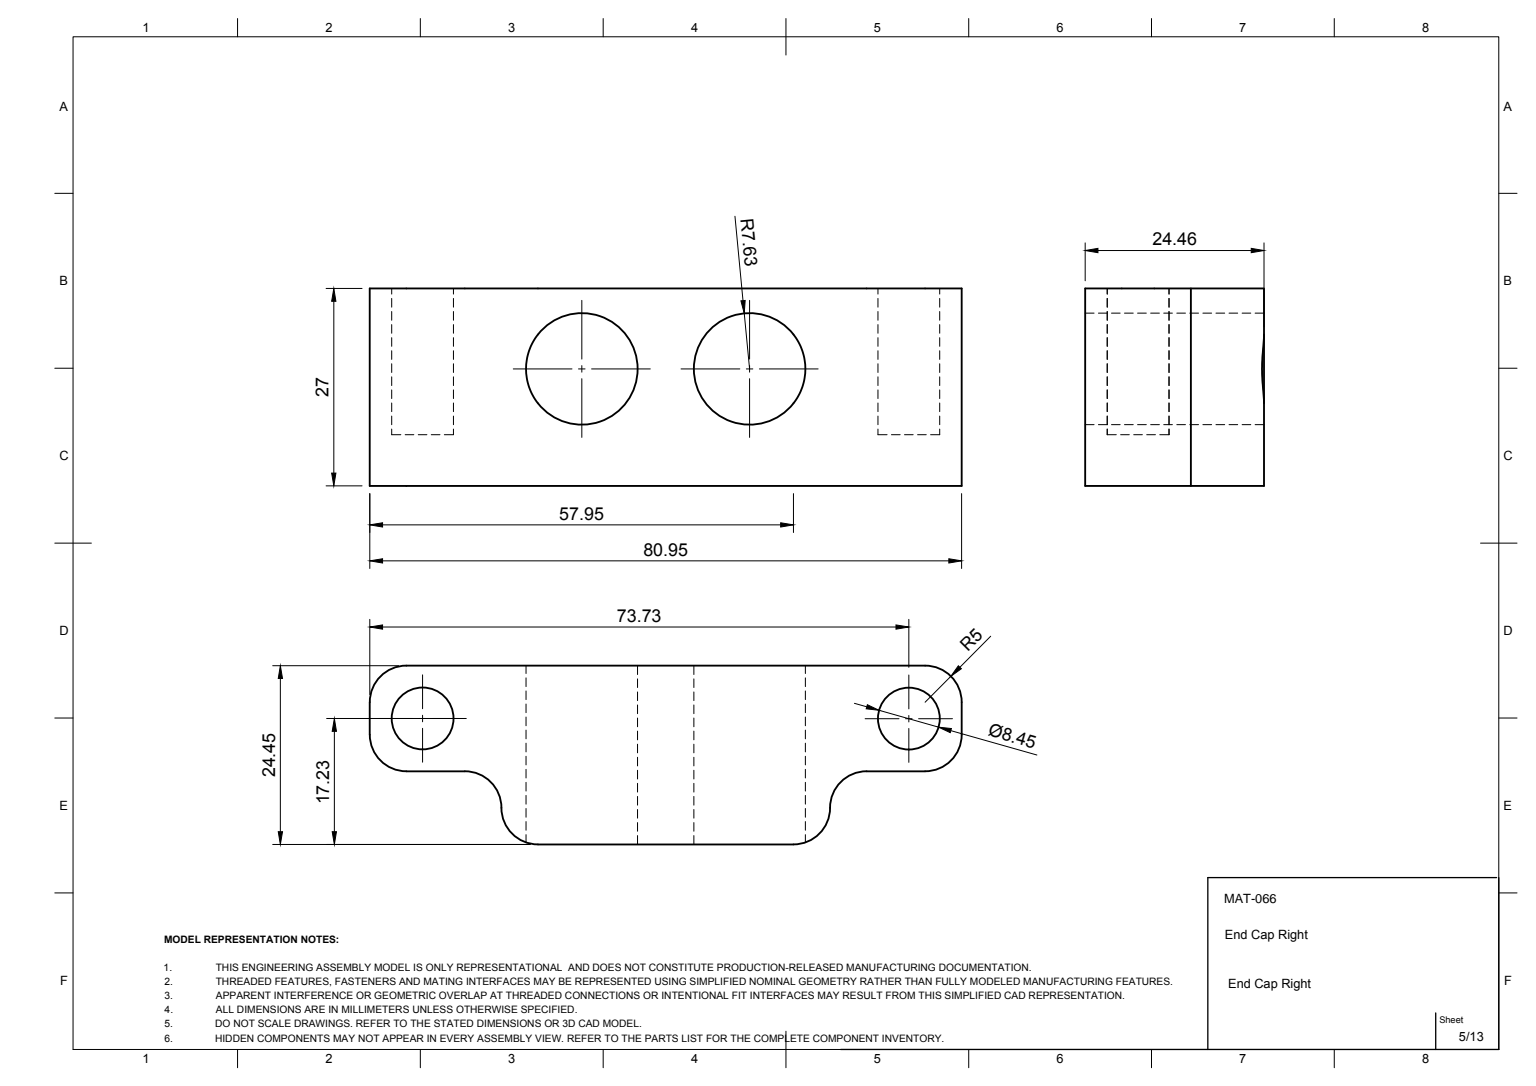
ISO-10303-21;
HEADER;
/* Generated by software containing ST-Developer
 * from STEP Tools, Inc. (www.steptools.com) 
 */

FILE_DESCRIPTION(
/* description */ ('CAx-IF Rec.Pracs.---Representation and Presentation of Product Manufa
cturing Information (PMI)---4.0---2014-10-13'),
/* implementation_level */ '2;1');

FILE_NAME(
/* name */ 'End Cap Right.step',
/* time_stamp */ '2026-10-24T15:58:00-07:00',
/* author */ (''),
/* organization */ (''),
/* preprocessor_version */ 'ST-DEVELOPER v20.2',
/* originating_system */ 'Autodesk Translation Framework v15.17.0.0',
/* authorisation */ '');

FILE_SCHEMA (('AP242_MANAGED_MODEL_BASED_3D_ENGINEERING_MIM_LF { 1 0 10303 442 2 1 4 }'));
ENDSEC;

DATA;
#10=MECHANICAL_DESIGN_GEOMETRIC_PRESENTATION_REPRESENTATION('',(#131),#8944);
#113=SHAPE_REPRESENTATION_RELATIONSHIP('SRR','None',#8995,#122);
#122=ADVANCED_BREP_SHAPE_REPRESENTATION('',(#140),#8936);
#131=STYLED_ITEM('',(#9054),#140);
#140=MANIFOLD_SOLID_BREP('Body1',#5152);
#150=B_SPLINE_CURVE_WITH_KNOTS('',3,(#8654,#8655,#8656,#8657,#8658,#8659),
 .UNSPECIFIED.,.F.,.F.,(4,2,4),(3.46797062946804,3.66737221611079,3.95578831781598),
 .UNSPECIFIED.);
#151=B_SPLINE_CURVE_WITH_KNOTS('',3,(#8660,#8661,#8662,#8663,#8664,#8665),
 .UNSPECIFIED.,.F.,.F.,(4,2,4),(3.95578831781598,4.24420441952117,4.44360600616391),
 .UNSPECIFIED.);
#152=B_SPLINE_CURVE_WITH_KNOTS('',3,(#8668,#8669,#8670,#8671,#8672,#8673,
#8674,#8675,#8676,#8677),.UNSPECIFIED.,.F.,.F.,(4,2,2,2,4),(3.46797062946804,
3.66737221611078,3.95578831781597,4.24420441952117,4.44360600616391),
 .UNSPECIFIED.);
#205=CYLINDRICAL_SURFACE('',#5639,0.004225);
#206=CYLINDRICAL_SURFACE('',#5643,0.004225);
#207=CYLINDRICAL_SURFACE('',#5657,0.005);
#208=CYLINDRICAL_SURFACE('',#5658,0.005);
#209=CYLINDRICAL_SURFACE('',#5659,0.005);
#210=CYLINDRICAL_SURFACE('',#5660,0.005);
#211=CYLINDRICAL_SURFACE('',#5665,0.007625);
#212=CYLINDRICAL_SURFACE('',#5666,0.007625);
#213=CYLINDRICAL_SURFACE('',#5667,0.005);
#214=CYLINDRICAL_SURFACE('',#5668,0.005);
#215=CYLINDRICAL_SURFACE('',#5669,0.005);
#216=CYLINDRICAL_SURFACE('',#5670,0.005);
#284=FACE_BOUND('',#819,.T.);
#285=FACE_BOUND('',#820,.T.);
#286=FACE_BOUND('',#826,.T.);
#287=FACE_BOUND('',#827,.T.);
#500=FACE_OUTER_BOUND('',#815,.T.);
#501=FACE_OUTER_BOUND('',#816,.T.);
#502=FACE_OUTER_BOUND('',#817,.T.);
#503=FACE_OUTER_BOUND('',#818,.T.);
#504=FACE_OUTER_BOUND('',#821,.T.);
#505=FACE_OUTER_BOUND('',#822,.T.);
#506=FACE_OUTER_BOUND('',#823,.T.);
#507=FACE_OUTER_BOUND('',#824,.T.);
#508=FACE_OUTER_BOUND('',#825,.T.);
#509=FACE_OUTER_BOUND('',#828,.T.);
#510=FACE_OUTER_BOUND('',#829,.T.);
#511=FACE_OUTER_BOUND('',#830,.T.);
#512=FACE_OUTER_BOUND('',#831,.T.);
#513=FACE_OUTER_BOUND('',#832,.T.);
#514=FACE_OUTER_BOUND('',#833,.T.);
#515=FACE_OUTER_BOUND('',#834,.T.);
#516=FACE_OUTER_BOUND('',#835,.T.);
#517=FACE_OUTER_BOUND('',#836,.T.);
#518=FACE_OUTER_BOUND('',#837,.T.);
#519=FACE_OUTER_BOUND('',#838,.T.);
#520=FACE_OUTER_BOUND('',#839,.T.);
#521=FACE_OUTER_BOUND('',#840,.T.);
#815=EDGE_LOOP('',(#4403,#4404,#4405,#4406,#4407,#4408,#4409,#4410,#4411,
#4412,#4413,#4414,#4415,#4416));
#816=EDGE_LOOP('',(#4417,#4418,#4419,#4420));
#817=EDGE_LOOP('',(#4421,#4422,#4423,#4424));
#818=EDGE_LOOP('',(#4425,#4426,#4427,#4428));
#819=EDGE_LOOP('',(#4429));
#820=EDGE_LOOP('',(#4430));
#821=EDGE_LOOP('',(#4431,#4432,#4433,#4434));
#822=EDGE_LOOP('',(#4435,#4436,#4437,#4438));
#823=EDGE_LOOP('',(#4439,#4440,#4441,#4442));
#824=EDGE_LOOP('',(#4443,#4444,#4445,#4446));
#825=EDGE_LOOP('',(#4447,#4448,#4449,#4450,#4451,#4452,#4453,#4454,#4455,
#4456,#4457,#4458,#4459,#4460));
#826=EDGE_LOOP('',(#4461));
#827=EDGE_LOOP('',(#4462));
#828=EDGE_LOOP('',(#4463));
#829=EDGE_LOOP('',(#4464));
#830=EDGE_LOOP('',(#4465,#4466,#4467,#4468));
#831=EDGE_LOOP('',(#4469,#4470,#4471,#4472));
#832=EDGE_LOOP('',(#4473,#4474,#4475,#4476));
#833=EDGE_LOOP('',(#4477,#4478,#4479,#4480));
#834=EDGE_LOOP('',(#4481,#4482,#4483,#4484,#4485,#4486,#4487,#4488,#4489));
#835=EDGE_LOOP('',(#4490,#4491,#4492,#4493,#4494,#4495));
#836=EDGE_LOOP('',(#4496,#4497,#4498,#4499,#4500,#4501));
#837=EDGE_LOOP('',(#4502,#4503,#4504,#4505,#4506,#4507));
#838=EDGE_LOOP('',(#4508,#4509,#4510,#4511));
#839=EDGE_LOOP('',(#4512,#4513,#4514,#4515,#4516,#4517,#4518));
#840=EDGE_LOOP('',(#4519,#4520,#4521,#4522));
#1085=CIRCLE('',#5625,0.00500000000000005);
#1086=CIRCLE('',#5626,0.00500000000000002);
#1087=CIRCLE('',#5627,0.005);
#1088=CIRCLE('',#5628,0.005);
#1089=CIRCLE('',#5629,0.005);
#1090=CIRCLE('',#5630,0.00500000000000004);
#1091=CIRCLE('',#5631,0.005);
#1092=CIRCLE('',#5632,0.00500000000000002);
#1093=CIRCLE('',#5636,0.007625);
#1094=CIRCLE('',#5637,0.007625);
#1095=CIRCLE('',#5640,0.004225);
#1096=CIRCLE('',#5641,0.004225);
#1097=CIRCLE('',#5644,0.004225);
#1098=CIRCLE('',#5645,0.004225);
#1099=CIRCLE('',#5647,0.005);
#1100=CIRCLE('',#5648,0.005);
#1101=CIRCLE('',#5649,0.005);
#1102=CIRCLE('',#5650,0.005);
#1103=CIRCLE('',#5651,0.005);
#1104=CIRCLE('',#5652,0.005);
#1105=CIRCLE('',#5653,0.005);
#1106=CIRCLE('',#5654,0.005);
#1107=CIRCLE('',#5662,0.007625);
#1108=CIRCLE('',#5663,0.007625);
#1109=CIRCLE('',#5664,0.007625);
#1564=LINE('',#8548,#2019);
#1565=LINE('',#8552,#2020);
#1566=LINE('',#8556,#2021);
#1567=LINE('',#8560,#2022);
#1568=LINE('',#8566,#2023);
#1569=LINE('',#8571,#2024);
#1570=LINE('',#8575,#2025);
#1571=LINE('',#8576,#2026);
#1572=LINE('',#8577,#2027);
#1573=LINE('',#8580,#2028);
#1574=LINE('',#8582,#2029);
#1575=LINE('',#8583,#2030);
#1576=LINE('',#8586,#2031);
#1577=LINE('',#8588,#2032);
#1578=LINE('',#8589,#2033);
#1579=LINE('',#8596,#2034);
#1580=LINE('',#8598,#2035);
#1581=LINE('',#8599,#2036);
#1582=LINE('',#8604,#2037);
#1583=LINE('',#8608,#2038);
#1584=LINE('',#8610,#2039);
#1585=LINE('',#8611,#2040);
#1586=LINE('',#8616,#2041);
#1587=LINE('',#8621,#2042);
#1588=LINE('',#8640,#2043);
#1589=LINE('',#8643,#2044);
#1590=LINE('',#8645,#2045);
#1591=LINE('',#8650,#2046);
#1592=LINE('',#8653,#2047);
#1593=LINE('',#8667,#2048);
#1594=LINE('',#8679,#2049);
#1595=LINE('',#8682,#2050);
#2019=VECTOR('',#6943,0.01);
#2020=VECTOR('',#6946,0.01);
#2021=VECTOR('',#6949,0.01);
#2022=VECTOR('',#6952,0.01);
#2023=VECTOR('',#6957,0.01);
#2024=VECTOR('',#6962,0.01);
#2025=VECTOR('',#6965,1.);
#2026=VECTOR('',#6966,1.);
#2027=VECTOR('',#6967,1.);
#2028=VECTOR('',#6970,1.);
#2029=VECTOR('',#6971,1.);
#2030=VECTOR('',#6972,0.01);
#2031=VECTOR('',#6975,1.);
#2032=VECTOR('',#6976,1.);
#2033=VECTOR('',#6977,0.01);
#2034=VECTOR('',#6984,1.);
#2035=VECTOR('',#6985,1.);
#2036=VECTOR('',#6986,0.01);
#2037=VECTOR('',#6991,0.004225);
#2038=VECTOR('',#6996,1.);
#2039=VECTOR('',#6997,1.);
#2040=VECTOR('',#6998,0.01);
#2041=VECTOR('',#7003,0.004225);
#2042=VECTOR('',#7008,1.);
#2043=VECTOR('',#7039,0.01);
#2044=VECTOR('',#7042,1.);
#2045=VECTOR('',#7043,1.);
#2046=VECTOR('',#7048,0.01);
#2047=VECTOR('',#7051,0.007625);
#2048=VECTOR('',#7054,0.007625);
#2049=VECTOR('',#7057,0.01);
#2050=VECTOR('',#7062,0.01);
#2458=VERTEX_POINT('',#8544);
#2459=VERTEX_POINT('',#8545);
#2460=VERTEX_POINT('',#8547);
#2461=VERTEX_POINT('',#8549);
#2462=VERTEX_POINT('',#8551);
#2463=VERTEX_POINT('',#8553);
#2464=VERTEX_POINT('',#8555);
#2465=VERTEX_POINT('',#8557);
#2466=VERTEX_POINT('',#8559);
#2467=VERTEX_POINT('',#8561);
#2468=VERTEX_POINT('',#8563);
#2469=VERTEX_POINT('',#8565);
#2470=VERTEX_POINT('',#8567);
#2471=VERTEX_POINT('',#8569);
#2472=VERTEX_POINT('',#8573);
#2473=VERTEX_POINT('',#8574);
#2474=VERTEX_POINT('',#8579);
#2475=VERTEX_POINT('',#8581);
#2476=VERTEX_POINT('',#8585);
#2477=VERTEX_POINT('',#8587);
#2478=VERTEX_POINT('',#8590);
#2479=VERTEX_POINT('',#8592);
#2480=VERTEX_POINT('',#8595);
#2481=VERTEX_POINT('',#8597);
#2482=VERTEX_POINT('',#8601);
#2483=VERTEX_POINT('',#8603);
#2484=VERTEX_POINT('',#8607);
#2485=VERTEX_POINT('',#8609);
#2486=VERTEX_POINT('',#8613);
#2487=VERTEX_POINT('',#8615);
#2488=VERTEX_POINT('',#8619);
#2489=VERTEX_POINT('',#8620);
#2490=VERTEX_POINT('',#8622);
#2491=VERTEX_POINT('',#8629);
#2492=VERTEX_POINT('',#8639);
#2493=VERTEX_POINT('',#8641);
#2494=VERTEX_POINT('',#8644);
#2495=VERTEX_POINT('',#8646);
#2496=VERTEX_POINT('',#8648);
#2497=VERTEX_POINT('',#8652);
#3122=EDGE_CURVE('',#2458,#2459,#1085,.T.);
#3123=EDGE_CURVE('',#2459,#2460,#1564,.T.);
#3124=EDGE_CURVE('',#2460,#2461,#1086,.T.);
#3125=EDGE_CURVE('',#2461,#2462,#1565,.T.);
#3126=EDGE_CURVE('',#2462,#2463,#1087,.T.);
#3127=EDGE_CURVE('',#2463,#2464,#1566,.T.);
#3128=EDGE_CURVE('',#2464,#2465,#1088,.T.);
#3129=EDGE_CURVE('',#2465,#2466,#1567,.T.);
#3130=EDGE_CURVE('',#2466,#2467,#1089,.T.);
#3131=EDGE_CURVE('',#2467,#2468,#1090,.T.);
#3132=EDGE_CURVE('',#2468,#2469,#1568,.T.);
#3133=EDGE_CURVE('',#2469,#2470,#1091,.T.);
#3134=EDGE_CURVE('',#2470,#2471,#1092,.T.);
#3135=EDGE_CURVE('',#2471,#2458,#1569,.T.);
#3136=EDGE_CURVE('',#2472,#2473,#1570,.T.);
#3137=EDGE_CURVE('',#2458,#2473,#1571,.T.);
#3138=EDGE_CURVE('',#2472,#2471,#1572,.F.);
#3139=EDGE_CURVE('',#2474,#2463,#1573,.F.);
#3140=EDGE_CURVE('',#2474,#2475,#1574,.T.);
#3141=EDGE_CURVE('',#2475,#2464,#1575,.T.);
#3142=EDGE_CURVE('',#2476,#2461,#1576,.F.);
#3143=EDGE_CURVE('',#2477,#2476,#1577,.T.);
#3144=EDGE_CURVE('',#2477,#2462,#1578,.T.);
#3145=EDGE_CURVE('',#2478,#2478,#1093,.T.);
#3146=EDGE_CURVE('',#2479,#2479,#1094,.T.);
#3147=EDGE_CURVE('',#2480,#2459,#1579,.F.);
#3148=EDGE_CURVE('',#2481,#2480,#1580,.T.);
#3149=EDGE_CURVE('',#2481,#2460,#1581,.T.);
#3150=EDGE_CURVE('',#2482,#2482,#1095,.T.);
#3151=EDGE_CURVE('',#2482,#2483,#1582,.T.);
#3152=EDGE_CURVE('',#2483,#2483,#1096,.T.);
#3153=EDGE_CURVE('',#2484,#2465,#1583,.F.);
#3154=EDGE_CURVE('',#2484,#2485,#1584,.T.);
#3155=EDGE_CURVE('',#2485,#2466,#1585,.T.);
#3156=EDGE_CURVE('',#2486,#2486,#1097,.T.);
#3157=EDGE_CURVE('',#2486,#2487,#1586,.T.);
#3158=EDGE_CURVE('',#2487,#2487,#1098,.T.);
#3159=EDGE_CURVE('',#2488,#2489,#1587,.T.);
#3160=EDGE_CURVE('',#2490,#2488,#1099,.F.);
#3161=EDGE_CURVE('',#2485,#2490,#1100,.T.);
#3162=EDGE_CURVE('',#2475,#2484,#1101,.F.);
#3163=EDGE_CURVE('',#2477,#2474,#1102,.F.);
#3164=EDGE_CURVE('',#2481,#2476,#1103,.F.);
#3165=EDGE_CURVE('',#2473,#2480,#1104,.F.);
#3166=EDGE_CURVE('',#2491,#2472,#1105,.T.);
#3167=EDGE_CURVE('',#2489,#2491,#1106,.F.);
#3168=EDGE_CURVE('',#2492,#2468,#1588,.T.);
#3169=EDGE_CURVE('',#2492,#2493,#1107,.T.);
#3170=EDGE_CURVE('',#2488,#2493,#1589,.F.);
#3171=EDGE_CURVE('',#2494,#2489,#1590,.T.);
#3172=EDGE_CURVE('',#2494,#2495,#1108,.T.);
#3173=EDGE_CURVE('',#2495,#2496,#1109,.T.);
#3174=EDGE_CURVE('',#2496,#2469,#1591,.T.);
#3175=EDGE_CURVE('',#2479,#2497,#1592,.T.);
#3176=EDGE_CURVE('',#2493,#2497,#150,.T.);
#3177=EDGE_CURVE('',#2497,#2492,#151,.T.);
#3178=EDGE_CURVE('',#2478,#2495,#1593,.T.);
#3179=EDGE_CURVE('',#2496,#2494,#152,.T.);
#3180=EDGE_CURVE('',#2491,#2470,#1594,.T.);
#3181=EDGE_CURVE('',#2490,#2467,#1595,.T.);
#4403=ORIENTED_EDGE('',*,*,#3122,.T.);
#4404=ORIENTED_EDGE('',*,*,#3123,.T.);
#4405=ORIENTED_EDGE('',*,*,#3124,.T.);
#4406=ORIENTED_EDGE('',*,*,#3125,.T.);
#4407=ORIENTED_EDGE('',*,*,#3126,.T.);
#4408=ORIENTED_EDGE('',*,*,#3127,.T.);
#4409=ORIENTED_EDGE('',*,*,#3128,.T.);
#4410=ORIENTED_EDGE('',*,*,#3129,.T.);
#4411=ORIENTED_EDGE('',*,*,#3130,.T.);
#4412=ORIENTED_EDGE('',*,*,#3131,.T.);
#4413=ORIENTED_EDGE('',*,*,#3132,.T.);
#4414=ORIENTED_EDGE('',*,*,#3133,.T.);
#4415=ORIENTED_EDGE('',*,*,#3134,.T.);
#4416=ORIENTED_EDGE('',*,*,#3135,.T.);
#4417=ORIENTED_EDGE('',*,*,#3136,.T.);
#4418=ORIENTED_EDGE('',*,*,#3137,.F.);
#4419=ORIENTED_EDGE('',*,*,#3135,.F.);
#4420=ORIENTED_EDGE('',*,*,#3138,.F.);
#4421=ORIENTED_EDGE('',*,*,#3139,.F.);
#4422=ORIENTED_EDGE('',*,*,#3140,.T.);
#4423=ORIENTED_EDGE('',*,*,#3141,.T.);
#4424=ORIENTED_EDGE('',*,*,#3127,.F.);
#4425=ORIENTED_EDGE('',*,*,#3142,.F.);
#4426=ORIENTED_EDGE('',*,*,#3143,.F.);
#4427=ORIENTED_EDGE('',*,*,#3144,.T.);
#4428=ORIENTED_EDGE('',*,*,#3125,.F.);
#4429=ORIENTED_EDGE('',*,*,#3145,.F.);
#4430=ORIENTED_EDGE('',*,*,#3146,.F.);
#4431=ORIENTED_EDGE('',*,*,#3147,.F.);
#4432=ORIENTED_EDGE('',*,*,#3148,.F.);
#4433=ORIENTED_EDGE('',*,*,#3149,.T.);
#4434=ORIENTED_EDGE('',*,*,#3123,.F.);
#4435=ORIENTED_EDGE('',*,*,#3150,.F.);
#4436=ORIENTED_EDGE('',*,*,#3151,.T.);
#4437=ORIENTED_EDGE('',*,*,#3152,.T.);
#4438=ORIENTED_EDGE('',*,*,#3151,.F.);
#4439=ORIENTED_EDGE('',*,*,#3153,.F.);
#4440=ORIENTED_EDGE('',*,*,#3154,.T.);
#4441=ORIENTED_EDGE('',*,*,#3155,.T.);
#4442=ORIENTED_EDGE('',*,*,#3129,.F.);
#4443=ORIENTED_EDGE('',*,*,#3156,.F.);
#4444=ORIENTED_EDGE('',*,*,#3157,.T.);
#4445=ORIENTED_EDGE('',*,*,#3158,.T.);
#4446=ORIENTED_EDGE('',*,*,#3157,.F.);
#4447=ORIENTED_EDGE('',*,*,#3159,.F.);
#4448=ORIENTED_EDGE('',*,*,#3160,.F.);
#4449=ORIENTED_EDGE('',*,*,#3161,.F.);
#4450=ORIENTED_EDGE('',*,*,#3154,.F.);
#4451=ORIENTED_EDGE('',*,*,#3162,.F.);
#4452=ORIENTED_EDGE('',*,*,#3140,.F.);
#4453=ORIENTED_EDGE('',*,*,#3163,.F.);
#4454=ORIENTED_EDGE('',*,*,#3143,.T.);
#4455=ORIENTED_EDGE('',*,*,#3164,.F.);
#4456=ORIENTED_EDGE('',*,*,#3148,.T.);
#4457=ORIENTED_EDGE('',*,*,#3165,.F.);
#4458=ORIENTED_EDGE('',*,*,#3136,.F.);
#4459=ORIENTED_EDGE('',*,*,#3166,.F.);
#4460=ORIENTED_EDGE('',*,*,#3167,.F.);
#4461=ORIENTED_EDGE('',*,*,#3152,.F.);
#4462=ORIENTED_EDGE('',*,*,#3158,.F.);
#4463=ORIENTED_EDGE('',*,*,#3156,.T.);
#4464=ORIENTED_EDGE('',*,*,#3150,.T.);
#4465=ORIENTED_EDGE('',*,*,#3141,.F.);
#4466=ORIENTED_EDGE('',*,*,#3162,.T.);
#4467=ORIENTED_EDGE('',*,*,#3153,.T.);
#4468=ORIENTED_EDGE('',*,*,#3128,.F.);
#4469=ORIENTED_EDGE('',*,*,#3144,.F.);
#4470=ORIENTED_EDGE('',*,*,#3163,.T.);
#4471=ORIENTED_EDGE('',*,*,#3139,.T.);
#4472=ORIENTED_EDGE('',*,*,#3126,.F.);
#4473=ORIENTED_EDGE('',*,*,#3149,.F.);
#4474=ORIENTED_EDGE('',*,*,#3164,.T.);
#4475=ORIENTED_EDGE('',*,*,#3142,.T.);
#4476=ORIENTED_EDGE('',*,*,#3124,.F.);
#4477=ORIENTED_EDGE('',*,*,#3137,.T.);
#4478=ORIENTED_EDGE('',*,*,#3165,.T.);
#4479=ORIENTED_EDGE('',*,*,#3147,.T.);
#4480=ORIENTED_EDGE('',*,*,#3122,.F.);
#4481=ORIENTED_EDGE('',*,*,#3168,.F.);
#4482=ORIENTED_EDGE('',*,*,#3169,.T.);
#4483=ORIENTED_EDGE('',*,*,#3170,.F.);
#4484=ORIENTED_EDGE('',*,*,#3159,.T.);
#4485=ORIENTED_EDGE('',*,*,#3171,.F.);
#4486=ORIENTED_EDGE('',*,*,#3172,.T.);
#4487=ORIENTED_EDGE('',*,*,#3173,.T.);
#4488=ORIENTED_EDGE('',*,*,#3174,.T.);
#4489=ORIENTED_EDGE('',*,*,#3132,.F.);
#4490=ORIENTED_EDGE('',*,*,#3146,.T.);
#4491=ORIENTED_EDGE('',*,*,#3175,.T.);
#4492=ORIENTED_EDGE('',*,*,#3176,.F.);
#4493=ORIENTED_EDGE('',*,*,#3169,.F.);
#4494=ORIENTED_EDGE('',*,*,#3177,.F.);
#4495=ORIENTED_EDGE('',*,*,#3175,.F.);
#4496=ORIENTED_EDGE('',*,*,#3145,.T.);
#4497=ORIENTED_EDGE('',*,*,#3178,.T.);
#4498=ORIENTED_EDGE('',*,*,#3172,.F.);
#4499=ORIENTED_EDGE('',*,*,#3179,.F.);
#4500=ORIENTED_EDGE('',*,*,#3173,.F.);
#4501=ORIENTED_EDGE('',*,*,#3178,.F.);
#4502=ORIENTED_EDGE('',*,*,#3174,.F.);
#4503=ORIENTED_EDGE('',*,*,#3179,.T.);
#4504=ORIENTED_EDGE('',*,*,#3171,.T.);
#4505=ORIENTED_EDGE('',*,*,#3167,.T.);
#4506=ORIENTED_EDGE('',*,*,#3180,.T.);
#4507=ORIENTED_EDGE('',*,*,#3133,.F.);
#4508=ORIENTED_EDGE('',*,*,#3180,.F.);
#4509=ORIENTED_EDGE('',*,*,#3166,.T.);
#4510=ORIENTED_EDGE('',*,*,#3138,.T.);
#4511=ORIENTED_EDGE('',*,*,#3134,.F.);
#4512=ORIENTED_EDGE('',*,*,#3181,.F.);
#4513=ORIENTED_EDGE('',*,*,#3160,.T.);
#4514=ORIENTED_EDGE('',*,*,#3170,.T.);
#4515=ORIENTED_EDGE('',*,*,#3176,.T.);
#4516=ORIENTED_EDGE('',*,*,#3177,.T.);
#4517=ORIENTED_EDGE('',*,*,#3168,.T.);
#4518=ORIENTED_EDGE('',*,*,#3131,.F.);
#4519=ORIENTED_EDGE('',*,*,#3155,.F.);
#4520=ORIENTED_EDGE('',*,*,#3161,.T.);
#4521=ORIENTED_EDGE('',*,*,#3181,.T.);
#4522=ORIENTED_EDGE('',*,*,#3130,.F.);
#4849=PLANE('',#5624);
#4850=PLANE('',#5633);
#4851=PLANE('',#5634);
#4852=PLANE('',#5635);
#4853=PLANE('',#5638);
#4854=PLANE('',#5642);
#4855=PLANE('',#5646);
#4856=PLANE('',#5655);
#4857=PLANE('',#5656);
#4858=PLANE('',#5661);
#5073=ADVANCED_FACE('',(#500),#4849,.T.);
#5074=ADVANCED_FACE('',(#501),#4850,.T.);
#5075=ADVANCED_FACE('',(#502),#4851,.T.);
#5076=ADVANCED_FACE('',(#503,#284,#285),#4852,.F.);
#5077=ADVANCED_FACE('',(#504),#4853,.F.);
#5078=ADVANCED_FACE('',(#505),#205,.F.);
#5079=ADVANCED_FACE('',(#506),#4854,.T.);
#5080=ADVANCED_FACE('',(#507),#206,.F.);
#5081=ADVANCED_FACE('',(#508,#286,#287),#4855,.F.);
#5082=ADVANCED_FACE('',(#509),#4856,.F.);
#5083=ADVANCED_FACE('',(#510),#4857,.F.);
#5084=ADVANCED_FACE('',(#511),#207,.T.);
#5085=ADVANCED_FACE('',(#512),#208,.T.);
#5086=ADVANCED_FACE('',(#513),#209,.T.);
#5087=ADVANCED_FACE('',(#514),#210,.T.);
#5088=ADVANCED_FACE('',(#515),#4858,.T.);
#5089=ADVANCED_FACE('',(#516),#211,.F.);
#5090=ADVANCED_FACE('',(#517),#212,.F.);
#5091=ADVANCED_FACE('',(#518),#213,.T.);
#5092=ADVANCED_FACE('',(#519),#214,.F.);
#5093=ADVANCED_FACE('',(#520),#215,.T.);
#5094=ADVANCED_FACE('',(#521),#216,.F.);
#5152=CLOSED_SHELL('',(#5073,#5074,#5075,#5076,#5077,#5078,#5079,#5080,
#5081,#5082,#5083,#5084,#5085,#5086,#5087,#5088,#5089,#5090,#5091,#5092,
#5093,#5094));
#5623=AXIS2_PLACEMENT_3D('',#8542,#6937,#6938);
#5624=AXIS2_PLACEMENT_3D('',#8543,#6939,#6940);
#5625=AXIS2_PLACEMENT_3D('',#8546,#6941,#6942);
#5626=AXIS2_PLACEMENT_3D('',#8550,#6944,#6945);
#5627=AXIS2_PLACEMENT_3D('',#8554,#6947,#6948);
#5628=AXIS2_PLACEMENT_3D('',#8558,#6950,#6951);
#5629=AXIS2_PLACEMENT_3D('',#8562,#6953,#6954);
#5630=AXIS2_PLACEMENT_3D('',#8564,#6955,#6956);
#5631=AXIS2_PLACEMENT_3D('',#8568,#6958,#6959);
#5632=AXIS2_PLACEMENT_3D('',#8570,#6960,#6961);
#5633=AXIS2_PLACEMENT_3D('',#8572,#6963,#6964);
#5634=AXIS2_PLACEMENT_3D('',#8578,#6968,#6969);
#5635=AXIS2_PLACEMENT_3D('',#8584,#6973,#6974);
#5636=AXIS2_PLACEMENT_3D('',#8591,#6978,#6979);
#5637=AXIS2_PLACEMENT_3D('',#8593,#6980,#6981);
#5638=AXIS2_PLACEMENT_3D('',#8594,#6982,#6983);
#5639=AXIS2_PLACEMENT_3D('',#8600,#6987,#6988);
#5640=AXIS2_PLACEMENT_3D('',#8602,#6989,#6990);
#5641=AXIS2_PLACEMENT_3D('',#8605,#6992,#6993);
#5642=AXIS2_PLACEMENT_3D('',#8606,#6994,#6995);
#5643=AXIS2_PLACEMENT_3D('',#8612,#6999,#7000);
#5644=AXIS2_PLACEMENT_3D('',#8614,#7001,#7002);
#5645=AXIS2_PLACEMENT_3D('',#8617,#7004,#7005);
#5646=AXIS2_PLACEMENT_3D('',#8618,#7006,#7007);
#5647=AXIS2_PLACEMENT_3D('',#8623,#7009,#7010);
#5648=AXIS2_PLACEMENT_3D('',#8624,#7011,#7012);
#5649=AXIS2_PLACEMENT_3D('',#8625,#7013,#7014);
#5650=AXIS2_PLACEMENT_3D('',#8626,#7015,#7016);
#5651=AXIS2_PLACEMENT_3D('',#8627,#7017,#7018);
#5652=AXIS2_PLACEMENT_3D('',#8628,#7019,#7020);
#5653=AXIS2_PLACEMENT_3D('',#8630,#7021,#7022);
#5654=AXIS2_PLACEMENT_3D('',#8631,#7023,#7024);
#5655=AXIS2_PLACEMENT_3D('',#8632,#7025,#7026);
#5656=AXIS2_PLACEMENT_3D('',#8633,#7027,#7028);
#5657=AXIS2_PLACEMENT_3D('',#8634,#7029,#7030);
#5658=AXIS2_PLACEMENT_3D('',#8635,#7031,#7032);
#5659=AXIS2_PLACEMENT_3D('',#8636,#7033,#7034);
#5660=AXIS2_PLACEMENT_3D('',#8637,#7035,#7036);
#5661=AXIS2_PLACEMENT_3D('',#8638,#7037,#7038);
#5662=AXIS2_PLACEMENT_3D('',#8642,#7040,#7041);
#5663=AXIS2_PLACEMENT_3D('',#8647,#7044,#7045);
#5664=AXIS2_PLACEMENT_3D('',#8649,#7046,#7047);
#5665=AXIS2_PLACEMENT_3D('',#8651,#7049,#7050);
#5666=AXIS2_PLACEMENT_3D('',#8666,#7052,#7053);
#5667=AXIS2_PLACEMENT_3D('',#8678,#7055,#7056);
#5668=AXIS2_PLACEMENT_3D('',#8680,#7058,#7059);
#5669=AXIS2_PLACEMENT_3D('',#8681,#7060,#7061);
#5670=AXIS2_PLACEMENT_3D('',#8683,#7063,#7064);
#6937=DIRECTION('axis',(0.,0.,1.));
#6938=DIRECTION('refdir',(1.,0.,0.));
#6939=DIRECTION('center_axis',(1.,-1.34352275263155E-12,-2.55900709108327E-25));
#6940=DIRECTION('ref_axis',(1.34352275263155E-12,1.,-8.56382735160077E-17));
#6941=DIRECTION('center_axis',(1.,-1.34352275263155E-12,-2.55900709108327E-25));
#6942=DIRECTION('ref_axis',(-1.34352275263155E-12,-1.,-7.01978908408492E-15));
#6943=DIRECTION('',(1.34352275940781E-12,1.,-8.56382735160077E-17));
#6944=DIRECTION('center_axis',(1.,-1.34352275940781E-12,6.7760076773746E-21));
#6945=DIRECTION('ref_axis',(6.776017108621E-21,7.01978908408497E-15,-1.));
#6946=DIRECTION('',(-4.77281939087608E-22,8.56382735160077E-17,1.));
#6947=DIRECTION('center_axis',(1.,-1.33641732527395E-12,-2.55901399361619E-25));
#6948=DIRECTION('ref_axis',(1.33641732527395E-12,1.,-8.56382735160077E-17));
#6949=DIRECTION('',(-1.35150638374886E-12,-1.,8.56382735160077E-17));
#6950=DIRECTION('center_axis',(1.,-1.34352275940781E-12,6.7760076773746E-21));
#6951=DIRECTION('ref_axis',(-6.77602665492437E-21,-1.4125216441686E-14,
1.));
#6952=DIRECTION('',(4.23489977076173E-21,-6.74697642126694E-15,-1.));
#6953=DIRECTION('center_axis',(-1.,1.34352275940781E-12,2.55900709108327E-25));
#6954=DIRECTION('ref_axis',(-2.56015766077872E-25,-8.56382735160077E-17,
-1.));
#6955=DIRECTION('center_axis',(1.,-1.34352275940781E-12,-7.10542735785685E-15));
#6956=DIRECTION('ref_axis',(7.10542735785219E-15,-3.46707540529401E-15,
1.));
#6957=DIRECTION('',(9.69167893318796E-22,9.30874939302446E-16,-1.));
#6958=DIRECTION('center_axis',(1.,-1.35062817998915E-12,-2.55950555256775E-25));
#6959=DIRECTION('ref_axis',(-1.35062817998915E-12,-1.,-7.01978908408499E-15));
#6960=DIRECTION('center_axis',(-1.,1.34352275263155E-12,2.55900709108327E-25));
#6961=DIRECTION('ref_axis',(1.34352275263155E-12,1.,-8.56382735160077E-17));
#6962=DIRECTION('',(-2.56015784192876E-25,-8.56382735160077E-17,-1.));
#6963=DIRECTION('center_axis',(0.,-1.,8.57182693503055E-17));
#6964=DIRECTION('ref_axis',(0.,-8.57182693503055E-17,-1.));
#6965=DIRECTION('',(0.,-8.57182693503055E-17,-1.));
#6966=DIRECTION('',(-1.,0.,0.));
#6967=DIRECTION('',(-1.,0.,0.));
#6968=DIRECTION('center_axis',(0.,0.,1.));
#6969=DIRECTION('ref_axis',(-1.,0.,0.));
#6970=DIRECTION('',(-1.,0.,0.));
#6971=DIRECTION('',(0.,-1.,0.));
#6972=DIRECTION('',(1.,-1.34336985979644E-12,0.));
#6973=DIRECTION('center_axis',(0.,-1.,6.42887020127291E-17));
#6974=DIRECTION('ref_axis',(0.,-6.42887020127291E-17,-1.));
#6975=DIRECTION('',(-1.,0.,0.));
#6976=DIRECTION('',(0.,-6.42887020127291E-17,-1.));
#6977=DIRECTION('',(1.,-1.34336985979644E-12,0.));
#6978=DIRECTION('center_axis',(0.,1.,-6.42887020127291E-17));
#6979=DIRECTION('ref_axis',(0.,-6.42887020127291E-17,-1.));
#6980=DIRECTION('center_axis',(0.,1.,-6.42887020127291E-17));
#6981=DIRECTION('ref_axis',(0.,-6.42887020127291E-17,-1.));
#6982=DIRECTION('center_axis',(0.,0.,1.));
#6983=DIRECTION('ref_axis',(-1.,0.,0.));
#6984=DIRECTION('',(-1.,0.,0.));
#6985=DIRECTION('',(0.,-1.,0.));
#6986=DIRECTION('',(1.,-1.34336985979644E-12,0.));
#6987=DIRECTION('center_axis',(-1.,0.,0.));
#6988=DIRECTION('ref_axis',(0.,0.,-1.));
#6989=DIRECTION('center_axis',(-1.,0.,0.));
#6990=DIRECTION('ref_axis',(0.,0.,1.));
#6991=DIRECTION('',(-1.,0.,0.));
#6992=DIRECTION('center_axis',(-1.,0.,0.));
#6993=DIRECTION('ref_axis',(0.,0.,1.));
#6994=DIRECTION('center_axis',(0.,-1.,8.57182693503055E-17));
#6995=DIRECTION('ref_axis',(0.,-8.57182693503055E-17,-1.));
#6996=DIRECTION('',(-1.,0.,0.));
#6997=DIRECTION('',(0.,-8.57182693503055E-17,-1.));
#6998=DIRECTION('',(1.,-1.34336985979644E-12,0.));
#6999=DIRECTION('center_axis',(-1.,0.,0.));
#7000=DIRECTION('ref_axis',(0.,0.,-1.));
#7001=DIRECTION('center_axis',(-1.,0.,0.));
#7002=DIRECTION('ref_axis',(0.,0.,1.));
#7003=DIRECTION('',(-1.,0.,0.));
#7004=DIRECTION('center_axis',(-1.,0.,0.));
#7005=DIRECTION('ref_axis',(0.,0.,1.));
#7006=DIRECTION('center_axis',(1.,0.,0.));
#7007=DIRECTION('ref_axis',(0.,-1.,0.));
#7008=DIRECTION('',(0.,-8.57182693503055E-17,-1.));
#7009=DIRECTION('center_axis',(-1.,0.,0.));
#7010=DIRECTION('ref_axis',(0.,0.,1.));
#7011=DIRECTION('center_axis',(-1.,0.,0.));
#7012=DIRECTION('ref_axis',(0.,0.,1.));
#7013=DIRECTION('center_axis',(-1.,0.,0.));
#7014=DIRECTION('ref_axis',(0.,0.,1.));
#7015=DIRECTION('center_axis',(-1.,0.,0.));
#7016=DIRECTION('ref_axis',(0.,0.,1.));
#7017=DIRECTION('center_axis',(-1.,0.,0.));
#7018=DIRECTION('ref_axis',(0.,0.,1.));
#7019=DIRECTION('center_axis',(-1.,0.,0.));
#7020=DIRECTION('ref_axis',(0.,0.,1.));
#7021=DIRECTION('center_axis',(-1.,0.,0.));
#7022=DIRECTION('ref_axis',(0.,0.,1.));
#7023=DIRECTION('center_axis',(-1.,0.,0.));
#7024=DIRECTION('ref_axis',(0.,0.,1.));
#7025=DIRECTION('center_axis',(1.,0.,0.));
#7026=DIRECTION('ref_axis',(0.,-1.,0.));
#7027=DIRECTION('center_axis',(1.,0.,0.));
#7028=DIRECTION('ref_axis',(0.,-1.,0.));
#7029=DIRECTION('center_axis',(-1.,0.,0.));
#7030=DIRECTION('ref_axis',(0.,0.,-1.));
#7031=DIRECTION('center_axis',(1.,0.,0.));
#7032=DIRECTION('ref_axis',(0.,0.,1.));
#7033=DIRECTION('center_axis',(-1.,0.,0.));
#7034=DIRECTION('ref_axis',(0.,0.,-1.));
#7035=DIRECTION('center_axis',(1.,0.,0.));
#7036=DIRECTION('ref_axis',(0.,0.,1.));
#7037=DIRECTION('center_axis',(0.,-1.,8.57182693503055E-17));
#7038=DIRECTION('ref_axis',(-1.,0.,0.));
#7039=DIRECTION('',(1.,-1.34336985979644E-12,0.));
#7040=DIRECTION('center_axis',(0.,1.,-8.57182693503055E-17));
#7041=DIRECTION('ref_axis',(0.,-8.57182693503055E-17,-1.));
#7042=DIRECTION('',(-1.,0.,0.));
#7043=DIRECTION('',(-1.,0.,0.));
#7044=DIRECTION('center_axis',(0.,1.,-8.57182693503055E-17));
#7045=DIRECTION('ref_axis',(0.,-8.57182693503055E-17,-1.));
#7046=DIRECTION('center_axis',(0.,1.,-8.57182693503055E-17));
#7047=DIRECTION('ref_axis',(0.,-8.57182693503055E-17,-1.));
#7048=DIRECTION('',(1.,-1.34336985979644E-12,0.));
#7049=DIRECTION('center_axis',(0.,-1.,8.57182693503055E-17));
#7050=DIRECTION('ref_axis',(0.,-8.57182693503055E-17,-1.));
#7051=DIRECTION('',(0.,-1.,8.57182693503055E-17));
#7052=DIRECTION('center_axis',(0.,-1.,8.57182693503055E-17));
#7053=DIRECTION('ref_axis',(0.,-8.57182693503055E-17,-1.));
#7054=DIRECTION('',(0.,-1.,8.57182693503055E-17));
#7055=DIRECTION('center_axis',(1.,0.,0.));
#7056=DIRECTION('ref_axis',(0.,0.,1.));
#7057=DIRECTION('',(1.,-1.34336985979644E-12,0.));
#7058=DIRECTION('center_axis',(-1.,0.,0.));
#7059=DIRECTION('ref_axis',(0.,0.,-1.));
#7060=DIRECTION('center_axis',(-1.,0.,0.));
#7061=DIRECTION('ref_axis',(0.,0.,-1.));
#7062=DIRECTION('',(1.,-1.34336985979644E-12,0.));
#7063=DIRECTION('center_axis',(1.,0.,0.));
#7064=DIRECTION('ref_axis',(0.,0.,1.));
#8542=CARTESIAN_POINT('',(0.,0.,0.));
#8543=CARTESIAN_POINT('Origin',(0.0735500000002153,-0.0149750000000067,
0.02565));
#8544=CARTESIAN_POINT('',(0.0735500000002123,-0.0172000000000067,-0.00982499999999996));
#8545=CARTESIAN_POINT('',(0.073550000000219,-0.0122000000000067,-0.014825));
#8546=CARTESIAN_POINT('Origin',(0.073550000000219,-0.0122000000000066,-0.00982499999999993));
#8547=CARTESIAN_POINT('',(0.073550000000225,-0.00775000000000667,-0.014825));
#8548=CARTESIAN_POINT('',(0.073550000000219,-0.0122000000000067,-0.014825));
#8549=CARTESIAN_POINT('',(0.0735500000002317,-0.00275000000000667,-0.00982499999999996));
#8550=CARTESIAN_POINT('Origin',(0.073550000000225,-0.0077500000000067,-0.00982499999999995));
#8551=CARTESIAN_POINT('',(0.0735500000002317,-0.00275000000000663,0.061125));
#8552=CARTESIAN_POINT('',(0.0735500000002317,-0.00275000000000667,-0.00982499999999996));
#8553=CARTESIAN_POINT('',(0.073550000000225,-0.00775000000000667,0.066125));
#8554=CARTESIAN_POINT('Origin',(0.0735500000002251,-0.00775000000000667,
0.061125));
#8555=CARTESIAN_POINT('',(0.073550000000219,-0.0122000000000067,0.066125));
#8556=CARTESIAN_POINT('',(0.073550000000225,-0.00775000000000667,0.066125));
#8557=CARTESIAN_POINT('',(0.0735500000002123,-0.0172000000000066,0.061125));
#8558=CARTESIAN_POINT('Origin',(0.073550000000219,-0.0122000000000066,0.061125));
#8559=CARTESIAN_POINT('',(0.0735500000002123,-0.0172000000000067,0.053125));
#8560=CARTESIAN_POINT('',(0.0735500000002123,-0.0172000000000066,0.061125));
#8561=CARTESIAN_POINT('',(0.0735500000002056,-0.0222000000000067,0.048125));
#8562=CARTESIAN_POINT('Origin',(0.0735500000002056,-0.0222000000000067,
0.053125));
#8563=CARTESIAN_POINT('',(0.0735500000001988,-0.0272000000000067,0.0431250000000001));
#8564=CARTESIAN_POINT('Origin',(0.0735500000002055,-0.0222000000000067,
0.043125));
#8565=CARTESIAN_POINT('',(0.0735500000001988,-0.0272000000000067,0.00817500000000003));
#8566=CARTESIAN_POINT('',(0.0735500000001988,-0.0272000000000067,0.0431250000000001));
#8567=CARTESIAN_POINT('',(0.0735500000002056,-0.0222000000000067,0.00317500000000006));
#8568=CARTESIAN_POINT('Origin',(0.0735500000002056,-0.0222000000000067,
0.00817500000000006));
#8569=CARTESIAN_POINT('',(0.0735500000002123,-0.0172000000000067,-0.00182499999999996));
#8570=CARTESIAN_POINT('Origin',(0.0735500000002056,-0.0222000000000067,
-0.00182499999999996));
#8571=CARTESIAN_POINT('',(0.0735500000002123,-0.0172000000000067,-0.00182499999999996));
#8572=CARTESIAN_POINT('Origin',(0.06655,-0.0172,0.02565));
#8573=CARTESIAN_POINT('',(0.04655,-0.0172,-0.001825));
#8574=CARTESIAN_POINT('',(0.04655,-0.0172,-0.009825));
#8575=CARTESIAN_POINT('',(0.04655,-0.0172,0.02565));
#8576=CARTESIAN_POINT('',(0.04655,-0.0172,-0.009825));
#8577=CARTESIAN_POINT('',(0.06655,-0.0172,-0.001825));
#8578=CARTESIAN_POINT('Origin',(0.06655,-0.009975,0.066125));
#8579=CARTESIAN_POINT('',(0.04655,-0.00775,0.066125));
#8580=CARTESIAN_POINT('',(0.06855,-0.00775,0.066125));
#8581=CARTESIAN_POINT('',(0.04655,-0.0122,0.066125));
#8582=CARTESIAN_POINT('',(0.04655,-0.009975,0.066125));
#8583=CARTESIAN_POINT('',(0.068550000000219,-0.0122,0.066125));
#8584=CARTESIAN_POINT('Origin',(0.06655,-0.00275,0.02565));
#8585=CARTESIAN_POINT('',(0.04655,-0.00275,-0.009825));
#8586=CARTESIAN_POINT('',(0.06655,-0.00275,-0.009825));
#8587=CARTESIAN_POINT('',(0.04655,-0.00275,0.061125));
#8588=CARTESIAN_POINT('',(0.04655,-0.00275,0.02565));
#8589=CARTESIAN_POINT('',(0.0685500000002317,-0.00274999999999991,0.061125));
#8590=CARTESIAN_POINT('',(0.05755,-0.00275,0.0218));
#8591=CARTESIAN_POINT('Origin',(0.05755,-0.00275,0.014175));
#8592=CARTESIAN_POINT('',(0.05755,-0.00275,0.04475));
#8593=CARTESIAN_POINT('Origin',(0.05755,-0.00275,0.037125));
#8594=CARTESIAN_POINT('Origin',(0.06655,-0.009975,-0.014825));
#8595=CARTESIAN_POINT('',(0.04655,-0.0122,-0.014825));
#8596=CARTESIAN_POINT('',(0.06855,-0.0122,-0.014825));
#8597=CARTESIAN_POINT('',(0.04655,-0.00775,-0.014825));
#8598=CARTESIAN_POINT('',(0.04655,-0.009975,-0.014825));
#8599=CARTESIAN_POINT('',(0.068550000000225,-0.00774999999999995,-0.014825));
#8600=CARTESIAN_POINT('Origin',(0.06655,-0.009975,-0.0076));
#8601=CARTESIAN_POINT('',(0.06655,-0.009975,-0.003375));
#8602=CARTESIAN_POINT('Origin',(0.06655,-0.009975,-0.0076));
#8603=CARTESIAN_POINT('',(0.04655,-0.009975,-0.003375));
#8604=CARTESIAN_POINT('',(0.06655,-0.009975,-0.003375));
#8605=CARTESIAN_POINT('Origin',(0.04655,-0.009975,-0.0076));
#8606=CARTESIAN_POINT('Origin',(0.06655,-0.0172,0.02565));
#8607=CARTESIAN_POINT('',(0.04655,-0.0172,0.061125));
#8608=CARTESIAN_POINT('',(0.06655,-0.0172,0.061125));
#8609=CARTESIAN_POINT('',(0.04655,-0.0172,0.053125));
#8610=CARTESIAN_POINT('',(0.04655,-0.0172,0.02565));
#8611=CARTESIAN_POINT('',(0.0685500000002123,-0.0172,0.053125));
#8612=CARTESIAN_POINT('Origin',(0.06655,-0.01,0.0589));
#8613=CARTESIAN_POINT('',(0.06655,-0.01,0.063125));
#8614=CARTESIAN_POINT('Origin',(0.06655,-0.01,0.0589));
#8615=CARTESIAN_POINT('',(0.04655,-0.01,0.063125));
#8616=CARTESIAN_POINT('',(0.06655,-0.01,0.063125));
#8617=CARTESIAN_POINT('Origin',(0.04655,-0.01,0.0589));
#8618=CARTESIAN_POINT('Origin',(0.04655,0.,0.02565));
#8619=CARTESIAN_POINT('',(0.04655,-0.0272,0.043125));
#8620=CARTESIAN_POINT('',(0.04655,-0.0272,0.008175));
#8621=CARTESIAN_POINT('',(0.04655,-0.0272,0.02565));
#8622=CARTESIAN_POINT('',(0.04655,-0.0222,0.048125));
#8623=CARTESIAN_POINT('Origin',(0.04655,-0.0222,0.043125));
#8624=CARTESIAN_POINT('Origin',(0.04655,-0.0222,0.053125));
#8625=CARTESIAN_POINT('Origin',(0.04655,-0.0122,0.061125));
#8626=CARTESIAN_POINT('Origin',(0.04655,-0.00775,0.061125));
#8627=CARTESIAN_POINT('Origin',(0.04655,-0.00775,-0.009825));
#8628=CARTESIAN_POINT('Origin',(0.04655,-0.0122,-0.009825));
#8629=CARTESIAN_POINT('',(0.04655,-0.0222,0.003175));
#8630=CARTESIAN_POINT('Origin',(0.04655,-0.0222,-0.001825));
#8631=CARTESIAN_POINT('Origin',(0.04655,-0.0222,0.008175));
#8632=CARTESIAN_POINT('Origin',(0.06655,-0.009975,0.02565));
#8633=CARTESIAN_POINT('Origin',(0.06655,-0.009975,0.02565));
#8634=CARTESIAN_POINT('Origin',(0.06655,-0.0122,0.061125));
#8635=CARTESIAN_POINT('Origin',(0.06655,-0.00775,0.061125));
#8636=CARTESIAN_POINT('Origin',(0.06655,-0.00775,-0.009825));
#8637=CARTESIAN_POINT('Origin',(0.06655,-0.0122,-0.009825));
#8638=CARTESIAN_POINT('Origin',(0.05755,-0.0272,0.02565));
#8639=CARTESIAN_POINT('',(0.0622553825561797,-0.0272,0.043125));
#8640=CARTESIAN_POINT('',(0.0685500000001988,-0.0272,0.0431250000000001));
#8641=CARTESIAN_POINT('',(0.0528446174438203,-0.0272,0.043125));
#8642=CARTESIAN_POINT('Origin',(0.05755,-0.0272,0.037125));
#8643=CARTESIAN_POINT('',(0.05755,-0.0272,0.043125));
#8644=CARTESIAN_POINT('',(0.0528446174438203,-0.0272,0.008175));
#8645=CARTESIAN_POINT('',(0.04655,-0.0272,0.008175));
#8646=CARTESIAN_POINT('',(0.05755,-0.0272,0.0218));
#8647=CARTESIAN_POINT('Origin',(0.05755,-0.0272,0.014175));
#8648=CARTESIAN_POINT('',(0.0622553825561797,-0.0272,0.008175));
#8649=CARTESIAN_POINT('Origin',(0.05755,-0.0272,0.014175));
#8650=CARTESIAN_POINT('',(0.0685500000001989,-0.0272,0.00817500000000003));
#8651=CARTESIAN_POINT('Origin',(0.05755,-0.0022,0.037125));
#8652=CARTESIAN_POINT('',(0.05755,-0.0269285700798444,0.04475));
#8653=CARTESIAN_POINT('',(0.05755,-0.0022,0.04475));
#8654=CARTESIAN_POINT('Ctrl Pts',(0.0528446174438203,-0.0272,0.043125));
#8655=CARTESIAN_POINT('Ctrl Pts',(0.0533814087034594,-0.0272,0.0435459680382359));
#8656=CARTESIAN_POINT('Ctrl Pts',(0.0539899057191737,-0.027146490983882,
0.0439040351600042));
#8657=CARTESIAN_POINT('Ctrl Pts',(0.0555707240629267,-0.0270066019492738,
0.0445577665669935));
#8658=CARTESIAN_POINT('Ctrl Pts',(0.056588612994316,-0.0269285700798444,
0.04475));
#8659=CARTESIAN_POINT('Ctrl Pts',(0.05755,-0.0269285700798444,0.04475));
#8660=CARTESIAN_POINT('Ctrl Pts',(0.05755,-0.0269285700798444,0.04475));
#8661=CARTESIAN_POINT('Ctrl Pts',(0.058511387005684,-0.0269285700798444,
0.04475));
#8662=CARTESIAN_POINT('Ctrl Pts',(0.0595292759370733,-0.0270066019492738,
0.0445577665669935));
#8663=CARTESIAN_POINT('Ctrl Pts',(0.0611100942808263,-0.027146490983882,
0.0439040351600042));
#8664=CARTESIAN_POINT('Ctrl Pts',(0.0617185912965407,-0.0272,0.0435459680382359));
#8665=CARTESIAN_POINT('Ctrl Pts',(0.0622553825561797,-0.0272,0.043125));
#8666=CARTESIAN_POINT('Origin',(0.05755,-0.0022,0.014175));
#8667=CARTESIAN_POINT('',(0.05755,-0.0022,0.0218));
#8668=CARTESIAN_POINT('Ctrl Pts',(0.0622553825561797,-0.0272,0.00817500000000001));
#8669=CARTESIAN_POINT('Ctrl Pts',(0.0617185912965407,-0.0272,0.00775403196176415));
#8670=CARTESIAN_POINT('Ctrl Pts',(0.0611100942808263,-0.027146490983882,
0.00739596483999584));
#8671=CARTESIAN_POINT('Ctrl Pts',(0.0595292759370733,-0.0270066019492738,
0.00674223343300649));
#8672=CARTESIAN_POINT('Ctrl Pts',(0.058511387005684,-0.0269285700798444,
0.00655));
#8673=CARTESIAN_POINT('Ctrl Pts',(0.056588612994316,-0.0269285700798444,
0.00655));
#8674=CARTESIAN_POINT('Ctrl Pts',(0.0555707240629267,-0.0270066019492738,
0.00674223343300649));
#8675=CARTESIAN_POINT('Ctrl Pts',(0.0539899057191737,-0.027146490983882,
0.00739596483999584));
#8676=CARTESIAN_POINT('Ctrl Pts',(0.0533814087034593,-0.0272,0.00775403196176414));
#8677=CARTESIAN_POINT('Ctrl Pts',(0.0528446174438203,-0.0272,0.00817500000000001));
#8678=CARTESIAN_POINT('Origin',(0.05755,-0.0222,0.008175));
#8679=CARTESIAN_POINT('',(0.0685500000002056,-0.0222,0.00317500000000006));
#8680=CARTESIAN_POINT('Origin',(0.05755,-0.0222,-0.001825));
#8681=CARTESIAN_POINT('Origin',(0.05755,-0.0222,0.043125));
#8682=CARTESIAN_POINT('',(0.0685500000002056,-0.0222,0.048125));
#8683=CARTESIAN_POINT('Origin',(0.06655,-0.0222,0.053125));
#8924=UNCERTAINTY_MEASURE_WITH_UNIT(LENGTH_MEASURE(1.E-5),#8945,
'DISTANCE_ACCURACY_VALUE',
'Maximum model space distance between geometric entities at asserted c
onnectivities');
#8932=UNCERTAINTY_MEASURE_WITH_UNIT(LENGTH_MEASURE(1.E-5),#8945,
'DISTANCE_ACCURACY_VALUE',
'Maximum model space distance between geometric entities at asserted c
onnectivities');
#8936=(
GEOMETRIC_REPRESENTATION_CONTEXT(3)
GLOBAL_UNCERTAINTY_ASSIGNED_CONTEXT((#8924))
GLOBAL_UNIT_ASSIGNED_CONTEXT((#8945,#8946,#8947))
REPRESENTATION_CONTEXT('','3D')
);
#8944=(
GEOMETRIC_REPRESENTATION_CONTEXT(3)
GLOBAL_UNCERTAINTY_ASSIGNED_CONTEXT((#8932))
GLOBAL_UNIT_ASSIGNED_CONTEXT((#8945,#8946,#8947))
REPRESENTATION_CONTEXT('','3D')
);
#8945=(
LENGTH_UNIT()
NAMED_UNIT(*)
SI_UNIT($,.METRE.)
);
#8946=(
NAMED_UNIT(*)
PLANE_ANGLE_UNIT()
SI_UNIT($,.RADIAN.)
);
#8947=(
NAMED_UNIT(*)
SI_UNIT($,.STERADIAN.)
SOLID_ANGLE_UNIT()
);
#8951=SHAPE_DEFINITION_REPRESENTATION(#8962,#8995);
#8962=PRODUCT_DEFINITION_SHAPE('',$,#9007);
#8995=SHAPE_REPRESENTATION('',(#5623),#8936);
#9003=PRODUCT_DEFINITION_CONTEXT('part definition',#9038,'design');
#9007=PRODUCT_DEFINITION('End Cap Right','End Cap Right',#9018,#9003);
#9018=PRODUCT_DEFINITION_FORMATION('',$,#9043);
#9038=APPLICATION_CONTEXT('Managed model based 3d engineering');
#9039=PRODUCT_CONTEXT('part definition',#9038,'mechanical');
#9043=PRODUCT('End Cap Right','End Cap Right',
'LEGAL AND USAGE DISCLAIMER: this Data/Model is provided \X2\201C\X0\A
S IS\X2\201D\X0\ for informational and representational only. It is a 
geometric approximation and is NOT engineered, certified, or guarantee
d for dimensional accuracy, exact tolerances, or production-level prec
ision. Vendor disclaims all implied warranties including fitness for a
 particular purpose. DO NOT USE FOR DIRECT PHYSICAL MANUFACTURING, AUT
OMATED PRODUCTION, OR SAFETY-CRITICAL SYSTEMS without independent engi
neering verification and resolution of any design discrepancies.',(#9039));
#9054=PRESENTATION_STYLE_ASSIGNMENT((#9059));
#9059=SURFACE_STYLE_USAGE(.BOTH.,#9064);
#9064=SURFACE_SIDE_STYLE('',(#9069));
#9069=SURFACE_STYLE_FILL_AREA(#9074);
#9074=FILL_AREA_STYLE('Opaque(137,137,137)',(#9079));
#9079=FILL_AREA_STYLE_COLOUR('Opaque(137,137,137)',#9084);
#9084=COLOUR_RGB('Opaque(137,137,137)',0.537254901960784,0.537254901960784,
0.537254901960784);
ENDSEC;
END-ISO-10303-21;
